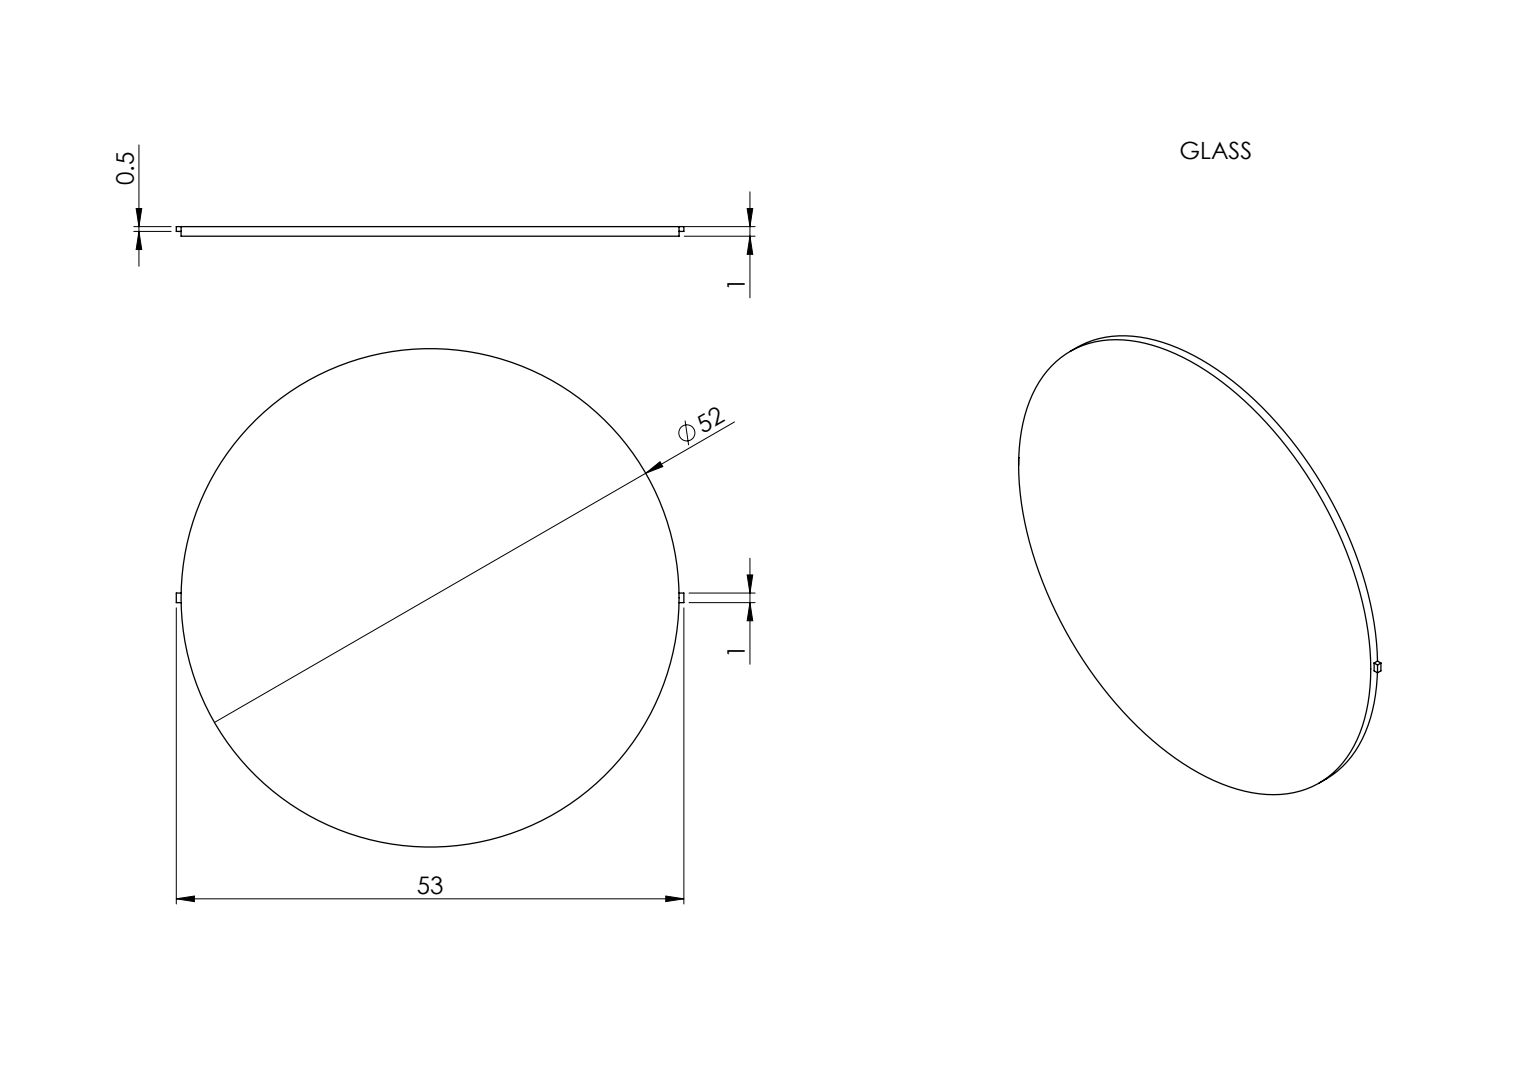
ISO-10303-21;
HEADER;
FILE_DESCRIPTION (('STEP AP214'),
    '1' );
FILE_NAME ('glass.step',
    '2026-10-26T12:50:16',
    ( '' ),
    ( '' ),
    'SwSTEP 2.0',
    'SolidWorks 2026',
    '' );
FILE_SCHEMA (( 'AUTOMOTIVE_DESIGN' ));
ENDSEC;

DATA;
#165=DIRECTION ( 'NONE',  ( -1.000000000000000000, 0.000000000000000000, 0.000000000000000000 ) ) ;
#175=LINE ( 'NONE', #12048, #20896 ) ;
#192=DIRECTION ( 'NONE',  ( 1.000000000000000000, -0.000000000000000000, -0.000000000000000000 ) ) ;
#288=ORIENTED_EDGE ( 'NONE', *, *, #23099, .T. ) ;
#324=DIRECTION ( 'NONE',  ( 0.000000000000000000, 0.000000000000000000, 1.000000000000000000 ) ) ;
#385=PLANE ( 'NONE',  #17255 ) ;
#447=LINE ( 'NONE', #10230, #15448 ) ;
#469=PRODUCT_DEFINITION_SHAPE ( 'NONE', 'NONE',  #20341 ) ;
#537=CARTESIAN_POINT ( 'NONE',  ( 0.000000000000000000, 0.000000000000000000, 19.50000000000000000 ) ) ;
#545=EDGE_LOOP ( 'NONE', ( #9181, #12765, #6775, #14139, #18806, #21870, #16789, #2419 ) ) ;
#649=EDGE_CURVE ( 'NONE', #12662, #14524, #9982, .T. ) ;
#747=FACE_OUTER_BOUND ( 'NONE', #11528, .T. ) ;
#913=CARTESIAN_POINT ( 'NONE',  ( 0.000000000000000000, 0.000000000000000000, 19.50000000000000000 ) ) ;
#940=CARTESIAN_POINT ( 'NONE',  ( 26.00000000000000711, 3.184081677783118980E-15, 20.00000000000000000 ) ) ;
#1040=UNCERTAINTY_MEASURE_WITH_UNIT (LENGTH_MEASURE( 1.000000000000000082E-05 ), #9039, 'distance_accuracy_value', 'NONE');
#1120=SHAPE_REPRESENTATION ( 'glass', ( #21036 ), #9344 ) ;
#1143=VERTEX_POINT ( 'NONE', #18649 ) ;
#1293=FACE_OUTER_BOUND ( 'NONE', #4147, .T. ) ;
#1406=ORIENTED_EDGE ( 'NONE', *, *, #3935, .F. ) ;
#1449=DIRECTION ( 'NONE',  ( 1.000000000000000000, 0.000000000000000000, 0.000000000000000000 ) ) ;
#1471=ADVANCED_FACE ( 'NONE', ( #20804 ), #3026, .T. ) ;
#1490=VECTOR ( 'NONE', #192, 1000.000000000000000 ) ;
#1528=VERTEX_POINT ( 'NONE', #940 ) ;
#1675=VECTOR ( 'NONE', #6954, 1000.000000000000000 ) ;
#1798=EDGE_CURVE ( 'NONE', #14524, #18045, #15690, .T. ) ;
#1814=DIRECTION ( 'NONE',  ( 1.000000000000000000, 0.000000000000000000, 0.000000000000000000 ) ) ;
#1866=ORIENTED_EDGE ( 'NONE', *, *, #3698, .F. ) ;
#1987=ORIENTED_EDGE ( 'NONE', *, *, #23515, .F. ) ;
#1995=AXIS2_PLACEMENT_3D ( 'NONE', #7561, #7812, #17496 ) ;
#2025=DIRECTION ( 'NONE',  ( 0.000000000000000000, 0.000000000000000000, -1.000000000000000000 ) ) ;
#2132=DIRECTION ( 'NONE',  ( -0.000000000000000000, -0.000000000000000000, -1.000000000000000000 ) ) ;
#2291=CARTESIAN_POINT ( 'NONE',  ( -26.50000000000000355, -0.5000000000000000000, 19.50000000000000000 ) ) ;
#2344=CARTESIAN_POINT ( 'NONE',  ( 26.49999999999999645, -0.5000000000000000000, 19.50000000000000000 ) ) ;
#2419=ORIENTED_EDGE ( 'NONE', *, *, #19939, .T. ) ;
#2431=CARTESIAN_POINT ( 'NONE',  ( 26.49999999999999645, -0.5000000000000000000, 19.50000000000000000 ) ) ;
#2446=FACE_OUTER_BOUND ( 'NONE', #24906, .T. ) ;
#2562=CARTESIAN_POINT ( 'NONE',  ( -25.99519186311192342, -0.5000000000000000000, 20.00000000000000000 ) ) ;
#2641=DIRECTION ( 'NONE',  ( 0.000000000000000000, 0.000000000000000000, -1.000000000000000000 ) ) ;
#2708=PLANE ( 'NONE',  #24311 ) ;
#2748=EDGE_LOOP ( 'NONE', ( #1866, #288, #10492, #1406 ) ) ;
#2946=ORIENTED_EDGE ( 'NONE', *, *, #3698, .T. ) ;
#2961=AXIS2_PLACEMENT_3D ( 'NONE', #23328, #5419, #13403 ) ;
#3026=PLANE ( 'NONE',  #8587 ) ;
#3046=ORIENTED_EDGE ( 'NONE', *, *, #23099, .F. ) ;
#3127=PRODUCT_DEFINITION_CONTEXT ( 'detailed design', #17969, 'design' ) ;
#3309=ADVANCED_FACE ( 'NONE', ( #15355 ), #17448, .T. ) ;
#3357=DIRECTION ( 'NONE',  ( 1.000000000000000000, -0.000000000000000000, -0.000000000000000000 ) ) ;
#3363=EDGE_LOOP ( 'NONE', ( #4654, #16710, #12568, #23853 ) ) ;
#3419=CIRCLE ( 'NONE', #21787, 26.00000000000000711 ) ;
#3496=COLOUR_RGB ( '',0.8941176470588234615, 0.8941176470588234615, 0.8941176470588234615 ) ;
#3606=EDGE_CURVE ( 'NONE', #12662, #13377, #25458, .T. ) ;
#3698=EDGE_CURVE ( 'NONE', #17369, #9796, #12489, .T. ) ;
#3751=APPLICATION_CONTEXT ( 'automotive_design' ) ;
#3754=LINE ( 'NONE', #23759, #24633 ) ;
#3796=ADVANCED_BREP_SHAPE_REPRESENTATION ( '', ( #22081, #21036 ), #9344 ) ;
#3851=DIRECTION ( 'NONE',  ( -0.000000000000000000, -0.000000000000000000, -1.000000000000000000 ) ) ;
#3877=CARTESIAN_POINT ( 'NONE',  ( 26.49999999999999645, 0.5000000000000000000, 19.00000000000000000 ) ) ;
#3924=( NAMED_UNIT ( * ) SI_UNIT ( $, .STERADIAN. ) SOLID_ANGLE_UNIT ( ) );
#3935=EDGE_CURVE ( 'NONE', #9796, #25585, #21733, .T. ) ;
#3948=VERTEX_POINT ( 'NONE', #18206 ) ;
#3953=ORIENTED_EDGE ( 'NONE', *, *, #19939, .F. ) ;
#3965=CARTESIAN_POINT ( 'NONE',  ( -26.50000000000000355, -0.5000000000000000000, 19.50000000000000000 ) ) ;
#3987=LINE ( 'NONE', #7781, #11324 ) ;
#4024=LINE ( 'NONE', #24681, #14557 ) ;
#4088=EDGE_CURVE ( 'NONE', #12917, #3948, #6942, .T. ) ;
#4147=EDGE_LOOP ( 'NONE', ( #25523, #16815, #25214, #3046, #1987 ) ) ;
#4355=EDGE_CURVE ( 'NONE', #14319, #1528, #8453, .T. ) ;
#4397=AXIS2_PLACEMENT_3D ( 'NONE', #22487, #16493, #10978 ) ;
#4414=CARTESIAN_POINT ( 'NONE',  ( 0.000000000000000000, 0.000000000000000000, 20.00000000000000000 ) ) ;
#4416=VERTEX_POINT ( 'NONE', #15955 ) ;
#4426=PRODUCT ( 'glass', 'glass', '', ( #9094 ) ) ;
#4554=DIRECTION ( 'NONE',  ( 0.000000000000000000, 0.000000000000000000, 1.000000000000000000 ) ) ;
#4654=ORIENTED_EDGE ( 'NONE', *, *, #5596, .F. ) ;
#4710=ADVANCED_FACE ( 'NONE', ( #12925 ), #385, .T. ) ;
#4936=ADVANCED_FACE ( 'NONE', ( #14981 ), #5044, .T. ) ;
#5044=CYLINDRICAL_SURFACE ( 'NONE', #21856, 26.00000000000000711 ) ;
#5078=ORIENTED_EDGE ( 'NONE', *, *, #24234, .T. ) ;
#5195=DIRECTION ( 'NONE',  ( 0.000000000000000000, 1.000000000000000000, 0.000000000000000000 ) ) ;
#5419=DIRECTION ( 'NONE',  ( 0.000000000000000000, 0.000000000000000000, 1.000000000000000000 ) ) ;
#5518=ORIENTED_EDGE ( 'NONE', *, *, #22622, .F. ) ;
#5596=EDGE_CURVE ( 'NONE', #18495, #14524, #8497, .T. ) ;
#5615=CARTESIAN_POINT ( 'NONE',  ( -25.99519186311192342, -0.5000000000000000000, 19.50000000000000000 ) ) ;
#5698=EDGE_LOOP ( 'NONE', ( #23371, #24133, #23127, #7405 ) ) ;
#5735=EDGE_CURVE ( 'NONE', #18705, #18585, #20613, .T. ) ;
#5943=DIRECTION ( 'NONE',  ( -1.000000000000000000, 0.000000000000000000, 0.000000000000000000 ) ) ;
#6028=CARTESIAN_POINT ( 'NONE',  ( 0.000000000000000000, 0.000000000000000000, 19.00000000000000000 ) ) ;
#6198=EDGE_CURVE ( 'NONE', #1528, #14319, #20521, .T. ) ;
#6268=( NAMED_UNIT ( * ) PLANE_ANGLE_UNIT ( ) SI_UNIT ( $, .RADIAN. ) );
#6284=DIRECTION ( 'NONE',  ( 0.000000000000000000, 0.000000000000000000, 1.000000000000000000 ) ) ;
#6352=ORIENTED_EDGE ( 'NONE', *, *, #22188, .T. ) ;
#6462=DIRECTION ( 'NONE',  ( 0.000000000000000000, 0.000000000000000000, 1.000000000000000000 ) ) ;
#6503=DIRECTION ( 'NONE',  ( -0.000000000000000000, -0.000000000000000000, -1.000000000000000000 ) ) ;
#6582=VECTOR ( 'NONE', #13913, 1000.000000000000000 ) ;
#6674=CARTESIAN_POINT ( 'NONE',  ( 25.99519186311192342, 0.5000000000000000000, 20.00000000000000000 ) ) ;
#6748=DIRECTION ( 'NONE',  ( 0.000000000000000000, 0.000000000000000000, -1.000000000000000000 ) ) ;
#6763=DIRECTION ( 'NONE',  ( 0.000000000000000000, -0.000000000000000000, 1.000000000000000000 ) ) ;
#6775=ORIENTED_EDGE ( 'NONE', *, *, #15340, .T. ) ;
#6842=DIRECTION ( 'NONE',  ( 0.000000000000000000, 0.000000000000000000, 1.000000000000000000 ) ) ;
#6891=PLANE ( 'NONE',  #16754 ) ;
#6912=SURFACE_STYLE_USAGE ( .BOTH. , #15024 ) ;
#6917=DIRECTION ( 'NONE',  ( 1.000000000000000000, 0.000000000000000000, 0.000000000000000000 ) ) ;
#6942=LINE ( 'NONE', #6674, #16399 ) ;
#6954=DIRECTION ( 'NONE',  ( 1.000000000000000000, -0.000000000000000000, -0.000000000000000000 ) ) ;
#6964=FACE_OUTER_BOUND ( 'NONE', #545, .T. ) ;
#7023=ORIENTED_EDGE ( 'NONE', *, *, #8660, .F. ) ;
#7072=( NAMED_UNIT ( * ) SI_UNIT ( $, .STERADIAN. ) SOLID_ANGLE_UNIT ( ) );
#7172=VECTOR ( 'NONE', #22696, 1000.000000000000000 ) ;
#7218=CARTESIAN_POINT ( 'NONE',  ( -26.00000000000000711, 0.000000000000000000, 19.50000000000000000 ) ) ;
#7405=ORIENTED_EDGE ( 'NONE', *, *, #3606, .T. ) ;
#7449=DIRECTION ( 'NONE',  ( 0.000000000000000000, 0.000000000000000000, 1.000000000000000000 ) ) ;
#7510=EDGE_LOOP ( 'NONE', ( #9564, #14844, #17583, #10328, #2946, #5078, #10015, #14168 ) ) ;
#7542=DIRECTION ( 'NONE',  ( 0.000000000000000000, 0.000000000000000000, -1.000000000000000000 ) ) ;
#7561=CARTESIAN_POINT ( 'NONE',  ( 0.000000000000000000, 0.000000000000000000, 19.50000000000000000 ) ) ;
#7563=CARTESIAN_POINT ( 'NONE',  ( 26.49999999999999645, -0.5000000000000000000, 19.50000000000000000 ) ) ;
#7656=LINE ( 'NONE', #13666, #1675 ) ;
#7781=CARTESIAN_POINT ( 'NONE',  ( -26.50000000000000355, -0.5000000000000000000, 19.50000000000000000 ) ) ;
#7789=CARTESIAN_POINT ( 'NONE',  ( 26.49999999999999645, -0.5000000000000000000, 19.50000000000000000 ) ) ;
#7812=DIRECTION ( 'NONE',  ( 0.000000000000000000, -0.000000000000000000, 1.000000000000000000 ) ) ;
#7880=CARTESIAN_POINT ( 'NONE',  ( -26.50000000000000355, -0.5000000000000000000, 19.00000000000000000 ) ) ;
#8107=ORIENTED_EDGE ( 'NONE', *, *, #22188, .F. ) ;
#8179=LINE ( 'NONE', #16156, #7172 ) ;
#8237=DIRECTION ( 'NONE',  ( -1.000000000000000000, 0.000000000000000000, 0.000000000000000000 ) ) ;
#8297=DIRECTION ( 'NONE',  ( 1.000000000000000000, 0.000000000000000000, 0.000000000000000000 ) ) ;
#8306=AXIS2_PLACEMENT_3D ( 'NONE', #4414, #6503, #16329 ) ;
#8431=DIRECTION ( 'NONE',  ( 1.000000000000000000, 0.000000000000000000, 0.000000000000000000 ) ) ;
#8453=CIRCLE ( 'NONE', #15547, 26.00000000000000711 ) ;
#8474=CARTESIAN_POINT ( 'NONE',  ( 26.49999999999999645, 0.5000000000000000000, 19.50000000000000000 ) ) ;
#8497=LINE ( 'NONE', #22867, #21044 ) ;
#8516=CARTESIAN_POINT ( 'NONE',  ( 25.99519186311192342, -0.5000000000000000000, 20.00000000000000000 ) ) ;
#8587=AXIS2_PLACEMENT_3D ( 'NONE', #10469, #16765, #2641 ) ;
#8590=EDGE_CURVE ( 'NONE', #3948, #18495, #14736, .T. ) ;
#8644=DIRECTION ( 'NONE',  ( -0.000000000000000000, -0.000000000000000000, -1.000000000000000000 ) ) ;
#8660=EDGE_CURVE ( 'NONE', #10164, #4416, #24575, .T. ) ;
#8688=CARTESIAN_POINT ( 'NONE',  ( 26.49999999999999645, -0.5000000000000000000, 19.00000000000000000 ) ) ;
#8717=DIRECTION ( 'NONE',  ( 0.000000000000000000, -0.000000000000000000, 1.000000000000000000 ) ) ;
#8888=( NAMED_UNIT ( * ) SI_UNIT ( $, .STERADIAN. ) SOLID_ANGLE_UNIT ( ) );
#8946=ORIENTED_EDGE ( 'NONE', *, *, #25469, .F. ) ;
#9039=( LENGTH_UNIT ( ) NAMED_UNIT ( * ) SI_UNIT ( .MILLI., .METRE. ) );
#9094=PRODUCT_CONTEXT ( 'NONE', #3751, 'mechanical' ) ;
#9112=ORIENTED_EDGE ( 'NONE', *, *, #10025, .F. ) ;
#9181=ORIENTED_EDGE ( 'NONE', *, *, #24234, .F. ) ;
#9235=SHAPE_DEFINITION_REPRESENTATION ( #469, #1120 ) ;
#9344=( GEOMETRIC_REPRESENTATION_CONTEXT ( 3 ) GLOBAL_UNCERTAINTY_ASSIGNED_CONTEXT ( ( #20656 ) ) GLOBAL_UNIT_ASSIGNED_CONTEXT ( ( #24180, #6268, #3924 ) ) REPRESENTATION_CONTEXT ( 'NONE', 'WORKASPACE' ) );
#9564=ORIENTED_EDGE ( 'NONE', *, *, #11490, .F. ) ;
#9796=VERTEX_POINT ( 'NONE', #14422 ) ;
#9886=CARTESIAN_POINT ( 'NONE',  ( -26.50000000000000355, 0.5000000000000000000, 19.50000000000000000 ) ) ;
#9982=LINE ( 'NONE', #16020, #1490 ) ;
#10015=ORIENTED_EDGE ( 'NONE', *, *, #8660, .T. ) ;
#10025=EDGE_CURVE ( 'NONE', #4416, #1143, #10887, .T. ) ;
#10128=AXIS2_PLACEMENT_3D ( 'NONE', #6028, #6284, #20666 ) ;
#10164=VERTEX_POINT ( 'NONE', #21296 ) ;
#10230=CARTESIAN_POINT ( 'NONE',  ( 26.49999999999999645, 0.5000000000000000000, 19.50000000000000000 ) ) ;
#10300=DIRECTION ( 'NONE',  ( 0.000000000000000000, 0.000000000000000000, -1.000000000000000000 ) ) ;
#10307=LINE ( 'NONE', #17794, #23006 ) ;
#10328=ORIENTED_EDGE ( 'NONE', *, *, #23515, .T. ) ;
#10362=CARTESIAN_POINT ( 'NONE',  ( 0.000000000000000000, 0.000000000000000000, 20.00000000000000000 ) ) ;
#10413=CYLINDRICAL_SURFACE ( 'NONE', #8306, 26.00000000000000711 ) ;
#10469=CARTESIAN_POINT ( 'NONE',  ( 26.49999999999999645, -0.5000000000000000000, 19.50000000000000000 ) ) ;
#10492=ORIENTED_EDGE ( 'NONE', *, *, #24097, .T. ) ;
#10536=VECTOR ( 'NONE', #22491, 1000.000000000000000 ) ;
#10577=MECHANICAL_DESIGN_GEOMETRIC_PRESENTATION_REPRESENTATION('',(#18128),#13936);
#10876=DIRECTION ( 'NONE',  ( 1.000000000000000000, -0.000000000000000000, -0.000000000000000000 ) ) ;
#10887=CIRCLE ( 'NONE', #24258, 26.00000000000000711 ) ;
#10978=DIRECTION ( 'NONE',  ( 1.000000000000000000, 0.000000000000000000, 0.000000000000000000 ) ) ;
#11022=ADVANCED_FACE ( 'NONE', ( #747 ), #6891, .T. ) ;
#11084=ADVANCED_FACE ( 'NONE', ( #2446 ), #24933, .T. ) ;
#11088=FILL_AREA_STYLE_COLOUR ( '', #3496 ) ;
#11324=VECTOR ( 'NONE', #2025, 1000.000000000000000 ) ;
#11465=EDGE_LOOP ( 'NONE', ( #7023, #3953, #22917, #6352 ) ) ;
#11490=EDGE_CURVE ( 'NONE', #1528, #1143, #8179, .T. ) ;
#11528=EDGE_LOOP ( 'NONE', ( #24469, #13562, #15601, #25845 ) ) ;
#11558=ORIENTED_EDGE ( 'NONE', *, *, #6198, .F. ) ;
#11570=CARTESIAN_POINT ( 'NONE',  ( -25.99519186311192342, 0.5000000000000000000, 19.50000000000000000 ) ) ;
#11853=ORIENTED_EDGE ( 'NONE', *, *, #5596, .T. ) ;
#12048=CARTESIAN_POINT ( 'NONE',  ( -26.00000000000000711, 0.000000000000000000, 20.00000000000000000 ) ) ;
#12470=PLANE ( 'NONE',  #16804 ) ;
#12489=LINE ( 'NONE', #2562, #22999 ) ;
#12527=VECTOR ( 'NONE', #10876, 1000.000000000000000 ) ;
#12565=EDGE_LOOP ( 'NONE', ( #21356, #24196 ) ) ;
#12568=ORIENTED_EDGE ( 'NONE', *, *, #3606, .F. ) ;
#12653=DIRECTION ( 'NONE',  ( 0.000000000000000000, -0.000000000000000000, 1.000000000000000000 ) ) ;
#12662=VERTEX_POINT ( 'NONE', #25605 ) ;
#12765=ORIENTED_EDGE ( 'NONE', *, *, #3935, .T. ) ;
#12777=CARTESIAN_POINT ( 'NONE',  ( 26.49999999999999645, 0.5000000000000000000, 19.50000000000000000 ) ) ;
#12907=DIRECTION ( 'NONE',  ( 1.000000000000000000, 0.000000000000000000, -0.000000000000000000 ) ) ;
#12917=VERTEX_POINT ( 'NONE', #18155 ) ;
#12925=FACE_OUTER_BOUND ( 'NONE', #17560, .T. ) ;
#13026=CARTESIAN_POINT ( 'NONE',  ( 0.000000000000000000, 0.000000000000000000, 20.00000000000000000 ) ) ;
#13138=PRODUCT_DEFINITION_FORMATION_WITH_SPECIFIED_SOURCE ( 'ANY', '', #4426, .NOT_KNOWN. ) ;
#13223=DIRECTION ( 'NONE',  ( 1.000000000000000000, 0.000000000000000000, 0.000000000000000000 ) ) ;
#13295=AXIS2_PLACEMENT_3D ( 'NONE', #537, #18689, #16490 ) ;
#13314=EDGE_CURVE ( 'NONE', #13377, #18495, #7656, .T. ) ;
#13353=CARTESIAN_POINT ( 'NONE',  ( 0.000000000000000000, 0.000000000000000000, 0.000000000000000000 ) ) ;
#13377=VERTEX_POINT ( 'NONE', #24745 ) ;
#13383=LINE ( 'NONE', #25668, #16838 ) ;
#13392=VECTOR ( 'NONE', #21196, 1000.000000000000000 ) ;
#13403=DIRECTION ( 'NONE',  ( 1.000000000000000000, 0.000000000000000000, -0.000000000000000000 ) ) ;
#13560=DIRECTION ( 'NONE',  ( 0.000000000000000000, -1.000000000000000000, -0.000000000000000000 ) ) ;
#13562=ORIENTED_EDGE ( 'NONE', *, *, #20462, .T. ) ;
#13666=CARTESIAN_POINT ( 'NONE',  ( 26.49999999999999645, 0.5000000000000000000, 19.00000000000000000 ) ) ;
#13675=DIRECTION ( 'NONE',  ( 0.000000000000000000, 0.000000000000000000, -1.000000000000000000 ) ) ;
#13913=DIRECTION ( 'NONE',  ( 0.000000000000000000, 1.000000000000000000, 0.000000000000000000 ) ) ;
#13936=( GEOMETRIC_REPRESENTATION_CONTEXT ( 3 ) GLOBAL_UNCERTAINTY_ASSIGNED_CONTEXT ( ( #22754 ) ) GLOBAL_UNIT_ASSIGNED_CONTEXT ( ( #14774, #18950, #8888 ) ) REPRESENTATION_CONTEXT ( 'NONE', 'WORKASPACE' ) );
#14139=ORIENTED_EDGE ( 'NONE', *, *, #13314, .T. ) ;
#14146=CARTESIAN_POINT ( 'NONE',  ( 26.49999999999999645, -0.5000000000000000000, 19.00000000000000000 ) ) ;
#14168=ORIENTED_EDGE ( 'NONE', *, *, #10025, .T. ) ;
#14169=DIRECTION ( 'NONE',  ( 0.000000000000000000, 0.000000000000000000, -1.000000000000000000 ) ) ;
#14319=VERTEX_POINT ( 'NONE', #24418 ) ;
#14422=CARTESIAN_POINT ( 'NONE',  ( -25.99519186311192342, -0.5000000000000000000, 19.00000000000000000 ) ) ;
#14510=DIRECTION ( 'NONE',  ( 0.000000000000000000, -0.000000000000000000, 1.000000000000000000 ) ) ;
#14524=VERTEX_POINT ( 'NONE', #11570 ) ;
#14557=VECTOR ( 'NONE', #5195, 1000.000000000000000 ) ;
#14639=CLOSED_SHELL ( 'NONE', ( #4936, #19694, #3309, #20551, #4710, #11084, #11022, #1471, #14819, #19714, #24870, #24317 ) ) ;
#14662=ORIENTED_EDGE ( 'NONE', *, *, #5735, .T. ) ;
#14722=DIRECTION ( 'NONE',  ( -1.000000000000000000, 0.000000000000000000, 0.000000000000000000 ) ) ;
#14736=CIRCLE ( 'NONE', #10128, 26.00000000000000711 ) ;
#14774=( LENGTH_UNIT ( ) NAMED_UNIT ( * ) SI_UNIT ( .MILLI., .METRE. ) );
#14819=ADVANCED_FACE ( 'NONE', ( #1293 ), #19456, .T. ) ;
#14825=DIRECTION ( 'NONE',  ( 1.000000000000000000, 0.000000000000000000, -0.000000000000000000 ) ) ;
#14842=CARTESIAN_POINT ( 'NONE',  ( 0.000000000000000000, 0.000000000000000000, 19.00000000000000000 ) ) ;
#14844=ORIENTED_EDGE ( 'NONE', *, *, #4355, .F. ) ;
#14895=SHAPE_REPRESENTATION_RELATIONSHIP ( 'NONE' , 'NONE' ,  #1120, #3796 ) ;
#14981=FACE_OUTER_BOUND ( 'NONE', #18207, .T. ) ;
#15024=SURFACE_SIDE_STYLE ('',( #16871 ) ) ;
#15148=ORIENTED_EDGE ( 'NONE', *, *, #8590, .T. ) ;
#15172=CARTESIAN_POINT ( 'NONE',  ( -25.99519186311192342, 0.5000000000000000000, 19.00000000000000000 ) ) ;
#15340=EDGE_CURVE ( 'NONE', #25585, #13377, #25799, .T. ) ;
#15355=FACE_OUTER_BOUND ( 'NONE', #12565, .T. ) ;
#15414=CARTESIAN_POINT ( 'NONE',  ( 26.49999999999999645, -0.5000000000000000000, 19.00000000000000000 ) ) ;
#15448=VECTOR ( 'NONE', #14169, 1000.000000000000000 ) ;
#15547=AXIS2_PLACEMENT_3D ( 'NONE', #23033, #7449, #1449 ) ;
#15569=ORIENTED_EDGE ( 'NONE', *, *, #22944, .F. ) ;
#15601=ORIENTED_EDGE ( 'NONE', *, *, #20281, .T. ) ;
#15690=CIRCLE ( 'NONE', #4397, 26.00000000000000711 ) ;
#15703=DIRECTION ( 'NONE',  ( 0.000000000000000000, 0.000000000000000000, 1.000000000000000000 ) ) ;
#15955=CARTESIAN_POINT ( 'NONE',  ( 25.99519186311192342, -0.5000000000000000000, 19.50000000000000000 ) ) ;
#16020=CARTESIAN_POINT ( 'NONE',  ( 26.49999999999999645, 0.5000000000000000000, 19.50000000000000000 ) ) ;
#16056=DIRECTION ( 'NONE',  ( -1.000000000000000000, 0.000000000000000000, 0.000000000000000000 ) ) ;
#16156=CARTESIAN_POINT ( 'NONE',  ( 26.00000000000000711, 3.184081677783118980E-15, 20.00000000000000000 ) ) ;
#16329=DIRECTION ( 'NONE',  ( -1.000000000000000000, 0.000000000000000000, 0.000000000000000000 ) ) ;
#16344=AXIS2_PLACEMENT_3D ( 'NONE', #16966, #6763, #12907 ) ;
#16399=VECTOR ( 'NONE', #8644, 1000.000000000000000 ) ;
#16451=VECTOR ( 'NONE', #6748, 1000.000000000000000 ) ;
#16459=FACE_OUTER_BOUND ( 'NONE', #3363, .T. ) ;
#16474=EDGE_CURVE ( 'NONE', #24372, #12662, #4024, .T. ) ;
#16490=DIRECTION ( 'NONE',  ( 1.000000000000000000, 0.000000000000000000, 0.000000000000000000 ) ) ;
#16493=DIRECTION ( 'NONE',  ( 0.000000000000000000, -0.000000000000000000, 1.000000000000000000 ) ) ;
#16512=CARTESIAN_POINT ( 'NONE',  ( -26.50000000000000355, -0.5000000000000000000, 19.00000000000000000 ) ) ;
#16577=CARTESIAN_POINT ( 'NONE',  ( 26.49999999999999645, 0.5000000000000000000, 19.50000000000000000 ) ) ;
#16710=ORIENTED_EDGE ( 'NONE', *, *, #13314, .F. ) ;
#16733=PRESENTATION_STYLE_ASSIGNMENT (( #6912 ) ) ;
#16754=AXIS2_PLACEMENT_3D ( 'NONE', #8474, #20883, #8717 ) ;
#16765=DIRECTION ( 'NONE',  ( 0.000000000000000000, -1.000000000000000000, -0.000000000000000000 ) ) ;
#16789=ORIENTED_EDGE ( 'NONE', *, *, #25469, .T. ) ;
#16790=PLANE ( 'NONE',  #17133 ) ;
#16804=AXIS2_PLACEMENT_3D ( 'NONE', #2291, #24634, #324 ) ;
#16813=FACE_OUTER_BOUND ( 'NONE', #5698, .T. ) ;
#16815=ORIENTED_EDGE ( 'NONE', *, *, #649, .F. ) ;
#16838=VECTOR ( 'NONE', #25398, 1000.000000000000000 ) ;
#16871=SURFACE_STYLE_FILL_AREA ( #24445 ) ;
#16966=CARTESIAN_POINT ( 'NONE',  ( 0.000000000000000000, 0.000000000000000000, 19.50000000000000000 ) ) ;
#17038=ORIENTED_EDGE ( 'NONE', *, *, #20462, .F. ) ;
#17133=AXIS2_PLACEMENT_3D ( 'NONE', #22920, #6842, #14825 ) ;
#17156=CARTESIAN_POINT ( 'NONE',  ( 26.49999999999999645, -0.5000000000000000000, 19.50000000000000000 ) ) ;
#17255=AXIS2_PLACEMENT_3D ( 'NONE', #2344, #24555, #10300 ) ;
#17369=VERTEX_POINT ( 'NONE', #5615 ) ;
#17421=ORIENTED_EDGE ( 'NONE', *, *, #18449, .F. ) ;
#17448=PLANE ( 'NONE',  #2961 ) ;
#17496=DIRECTION ( 'NONE',  ( 1.000000000000000000, 0.000000000000000000, -0.000000000000000000 ) ) ;
#17533=STYLED_ITEM('',(#25900),#22081);
#17560=EDGE_LOOP ( 'NONE', ( #8946, #24612, #19493, #14662 ) ) ;
#17583=ORIENTED_EDGE ( 'NONE', *, *, #22622, .T. ) ;
#17737=PLANE ( 'NONE',  #22931 ) ;
#17757=CARTESIAN_POINT ( 'NONE',  ( 0.000000000000000000, 0.000000000000000000, 19.50000000000000000 ) ) ;
#17794=CARTESIAN_POINT ( 'NONE',  ( 26.49999999999999645, -0.5000000000000000000, 19.50000000000000000 ) ) ;
#17842=EDGE_CURVE ( 'NONE', #3948, #19738, #25330, .T. ) ;
#17882=DIRECTION ( 'NONE',  ( 0.000000000000000000, -0.000000000000000000, 1.000000000000000000 ) ) ;
#17969=APPLICATION_CONTEXT ( 'automotive_design' ) ;
#18045=VERTEX_POINT ( 'NONE', #7218 ) ;
#18128=STYLED_ITEM ( 'NONE', ( #16733 ), #3796 ) ;
#18138=CARTESIAN_POINT ( 'NONE',  ( 26.49999999999999645, 0.5000000000000000000, 19.00000000000000000 ) ) ;
#18155=CARTESIAN_POINT ( 'NONE',  ( 25.99519186311192342, 0.5000000000000000000, 19.50000000000000000 ) ) ;
#18177=ORIENTED_EDGE ( 'NONE', *, *, #1798, .T. ) ;
#18206=CARTESIAN_POINT ( 'NONE',  ( 25.99519186311192342, 0.5000000000000000000, 19.00000000000000000 ) ) ;
#18207=EDGE_LOOP ( 'NONE', ( #11558, #19024, #18765, #23685, #15148, #11853, #18177, #5518 ) ) ;
#18449=EDGE_CURVE ( 'NONE', #1143, #12917, #24559, .T. ) ;
#18495=VERTEX_POINT ( 'NONE', #15172 ) ;
#18585=VERTEX_POINT ( 'NONE', #15414 ) ;
#18649=CARTESIAN_POINT ( 'NONE',  ( 26.00000000000000711, 3.184081677783118980E-15, 19.50000000000000000 ) ) ;
#18689=DIRECTION ( 'NONE',  ( 0.000000000000000000, -0.000000000000000000, 1.000000000000000000 ) ) ;
#18705=VERTEX_POINT ( 'NONE', #7563 ) ;
#18765=ORIENTED_EDGE ( 'NONE', *, *, #18449, .T. ) ;
#18805=MECHANICAL_DESIGN_GEOMETRIC_PRESENTATION_REPRESENTATION('',(#17533),#22963);
#18806=ORIENTED_EDGE ( 'NONE', *, *, #8590, .F. ) ;
#18950=( NAMED_UNIT ( * ) PLANE_ANGLE_UNIT ( ) SI_UNIT ( $, .RADIAN. ) );
#19024=ORIENTED_EDGE ( 'NONE', *, *, #11490, .T. ) ;
#19456=PLANE ( 'NONE',  #1995 ) ;
#19493=ORIENTED_EDGE ( 'NONE', *, *, #22944, .T. ) ;
#19531=VECTOR ( 'NONE', #3357, 1000.000000000000000 ) ;
#19658=VECTOR ( 'NONE', #165, 1000.000000000000000 ) ;
#19694=ADVANCED_FACE ( 'NONE', ( #24541 ), #10413, .T. ) ;
#19714=ADVANCED_FACE ( 'NONE', ( #20072 ), #17737, .T. ) ;
#19738=VERTEX_POINT ( 'NONE', #18138 ) ;
#19939=EDGE_CURVE ( 'NONE', #18585, #10164, #24397, .T. ) ;
#20072=FACE_OUTER_BOUND ( 'NONE', #2748, .T. ) ;
#20079=CIRCLE ( 'NONE', #25526, 26.00000000000000711 ) ;
#20281=EDGE_CURVE ( 'NONE', #23846, #19738, #447, .T. ) ;
#20341=PRODUCT_DEFINITION ( 'UNKNOWN', '', #13138, #3127 ) ;
#20462=EDGE_CURVE ( 'NONE', #12917, #23846, #21211, .T. ) ;
#20521=CIRCLE ( 'NONE', #22189, 26.00000000000000711 ) ;
#20551=ADVANCED_FACE ( 'NONE', ( #6964 ), #16790, .F. ) ;
#20591=DIRECTION ( 'NONE',  ( 0.000000000000000000, 0.000000000000000000, 1.000000000000000000 ) ) ;
#20613=LINE ( 'NONE', #2431, #16451 ) ;
#20656=UNCERTAINTY_MEASURE_WITH_UNIT (LENGTH_MEASURE( 1.000000000000000082E-05 ), #24180, 'distance_accuracy_value', 'NONE');
#20666=DIRECTION ( 'NONE',  ( 1.000000000000000000, 0.000000000000000000, 0.000000000000000000 ) ) ;
#20804=FACE_OUTER_BOUND ( 'NONE', #11465, .T. ) ;
#20883=DIRECTION ( 'NONE',  ( 0.000000000000000000, 1.000000000000000000, 0.000000000000000000 ) ) ;
#20896=VECTOR ( 'NONE', #2132, 1000.000000000000000 ) ;
#21036=AXIS2_PLACEMENT_3D ( 'NONE', #13353, #15703, #13223 ) ;
#21044=VECTOR ( 'NONE', #4554, 1000.000000000000000 ) ;
#21196=DIRECTION ( 'NONE',  ( -0.000000000000000000, -1.000000000000000000, -0.000000000000000000 ) ) ;
#21211=LINE ( 'NONE', #22797, #12527 ) ;
#21285=VECTOR ( 'NONE', #14722, 1000.000000000000000 ) ;
#21296=CARTESIAN_POINT ( 'NONE',  ( 25.99519186311192342, -0.5000000000000000000, 19.00000000000000000 ) ) ;
#21356=ORIENTED_EDGE ( 'NONE', *, *, #4355, .T. ) ;
#21733=LINE ( 'NONE', #14146, #19658 ) ;
#21787=AXIS2_PLACEMENT_3D ( 'NONE', #14842, #20591, #8297 ) ;
#21856=AXIS2_PLACEMENT_3D ( 'NONE', #13026, #3851, #5943 ) ;
#21870=ORIENTED_EDGE ( 'NONE', *, *, #17842, .T. ) ;
#22081=MANIFOLD_SOLID_BREP ( 'Boss-Extrude2', #14639 ) ;
#22182=DIRECTION ( 'NONE',  ( -0.000000000000000000, -0.000000000000000000, -1.000000000000000000 ) ) ;
#22188=EDGE_CURVE ( 'NONE', #18705, #4416, #3754, .T. ) ;
#22189=AXIS2_PLACEMENT_3D ( 'NONE', #10362, #6462, #8431 ) ;
#22487=CARTESIAN_POINT ( 'NONE',  ( 0.000000000000000000, 0.000000000000000000, 19.50000000000000000 ) ) ;
#22491=DIRECTION ( 'NONE',  ( 0.000000000000000000, 0.000000000000000000, 1.000000000000000000 ) ) ;
#22622=EDGE_CURVE ( 'NONE', #14319, #18045, #175, .T. ) ;
#22696=DIRECTION ( 'NONE',  ( -0.000000000000000000, -0.000000000000000000, -1.000000000000000000 ) ) ;
#22754=UNCERTAINTY_MEASURE_WITH_UNIT (LENGTH_MEASURE( 1.000000000000000082E-05 ), #14774, 'distance_accuracy_value', 'NONE');
#22797=CARTESIAN_POINT ( 'NONE',  ( 26.49999999999999645, 0.5000000000000000000, 19.50000000000000000 ) ) ;
#22848=DIRECTION ( 'NONE',  ( 0.000000000000000000, 1.000000000000000000, 0.000000000000000000 ) ) ;
#22867=CARTESIAN_POINT ( 'NONE',  ( -25.99519186311192342, 0.5000000000000000000, 20.00000000000000000 ) ) ;
#22917=ORIENTED_EDGE ( 'NONE', *, *, #5735, .F. ) ;
#22920=CARTESIAN_POINT ( 'NONE',  ( 0.000000000000000000, 0.000000000000000000, 19.00000000000000000 ) ) ;
#22931=AXIS2_PLACEMENT_3D ( 'NONE', #7789, #13560, #13675 ) ;
#22944=EDGE_CURVE ( 'NONE', #23846, #18705, #25641, .T. ) ;
#22963=( GEOMETRIC_REPRESENTATION_CONTEXT ( 3 ) GLOBAL_UNCERTAINTY_ASSIGNED_CONTEXT ( ( #1040 ) ) GLOBAL_UNIT_ASSIGNED_CONTEXT ( ( #9039, #24987, #7072 ) ) REPRESENTATION_CONTEXT ( 'NONE', 'WORKASPACE' ) );
#22999=VECTOR ( 'NONE', #22182, 1000.000000000000000 ) ;
#23006=VECTOR ( 'NONE', #8237, 1000.000000000000000 ) ;
#23033=CARTESIAN_POINT ( 'NONE',  ( 0.000000000000000000, 0.000000000000000000, 20.00000000000000000 ) ) ;
#23099=EDGE_CURVE ( 'NONE', #17369, #24372, #10307, .T. ) ;
#23127=ORIENTED_EDGE ( 'NONE', *, *, #16474, .T. ) ;
#23328=CARTESIAN_POINT ( 'NONE',  ( 0.000000000000000000, 0.000000000000000000, 20.00000000000000000 ) ) ;
#23371=ORIENTED_EDGE ( 'NONE', *, *, #15340, .F. ) ;
#23515=EDGE_CURVE ( 'NONE', #18045, #17369, #20079, .T. ) ;
#23685=ORIENTED_EDGE ( 'NONE', *, *, #4088, .T. ) ;
#23759=CARTESIAN_POINT ( 'NONE',  ( 26.49999999999999645, -0.5000000000000000000, 19.50000000000000000 ) ) ;
#23846=VERTEX_POINT ( 'NONE', #12777 ) ;
#23853=ORIENTED_EDGE ( 'NONE', *, *, #649, .T. ) ;
#24097=EDGE_CURVE ( 'NONE', #24372, #25585, #3987, .T. ) ;
#24133=ORIENTED_EDGE ( 'NONE', *, *, #24097, .F. ) ;
#24180=( LENGTH_UNIT ( ) NAMED_UNIT ( * ) SI_UNIT ( .MILLI., .METRE. ) );
#24196=ORIENTED_EDGE ( 'NONE', *, *, #6198, .T. ) ;
#24234=EDGE_CURVE ( 'NONE', #9796, #10164, #3419, .T. ) ;
#24258=AXIS2_PLACEMENT_3D ( 'NONE', #913, #14510, #6917 ) ;
#24311=AXIS2_PLACEMENT_3D ( 'NONE', #16577, #22848, #12653 ) ;
#24317=ADVANCED_FACE ( 'NONE', ( #16813 ), #12470, .T. ) ;
#24372=VERTEX_POINT ( 'NONE', #3965 ) ;
#24397=LINE ( 'NONE', #8688, #21285 ) ;
#24418=CARTESIAN_POINT ( 'NONE',  ( -26.00000000000000711, 0.000000000000000000, 20.00000000000000000 ) ) ;
#24445=FILL_AREA_STYLE ('',( #11088 ) ) ;
#24469=ORIENTED_EDGE ( 'NONE', *, *, #4088, .F. ) ;
#24541=FACE_OUTER_BOUND ( 'NONE', #7510, .T. ) ;
#24555=DIRECTION ( 'NONE',  ( 1.000000000000000000, -0.000000000000000000, 0.000000000000000000 ) ) ;
#24559=CIRCLE ( 'NONE', #13295, 26.00000000000000711 ) ;
#24575=LINE ( 'NONE', #8516, #10536 ) ;
#24612=ORIENTED_EDGE ( 'NONE', *, *, #20281, .F. ) ;
#24633=VECTOR ( 'NONE', #16056, 1000.000000000000000 ) ;
#24634=DIRECTION ( 'NONE',  ( -1.000000000000000000, 0.000000000000000000, 0.000000000000000000 ) ) ;
#24663=VECTOR ( 'NONE', #7542, 1000.000000000000000 ) ;
#24681=CARTESIAN_POINT ( 'NONE',  ( -26.50000000000000355, -0.5000000000000000000, 19.50000000000000000 ) ) ;
#24745=CARTESIAN_POINT ( 'NONE',  ( -26.50000000000000355, 0.5000000000000000000, 19.00000000000000000 ) ) ;
#24870=ADVANCED_FACE ( 'NONE', ( #16459 ), #2708, .T. ) ;
#24906=EDGE_LOOP ( 'NONE', ( #9112, #8107, #15569, #17038, #17421 ) ) ;
#24933=PLANE ( 'NONE',  #16344 ) ;
#24987=( NAMED_UNIT ( * ) PLANE_ANGLE_UNIT ( ) SI_UNIT ( $, .RADIAN. ) );
#25214=ORIENTED_EDGE ( 'NONE', *, *, #16474, .F. ) ;
#25330=LINE ( 'NONE', #3877, #19531 ) ;
#25398=DIRECTION ( 'NONE',  ( -0.000000000000000000, -1.000000000000000000, -0.000000000000000000 ) ) ;
#25458=LINE ( 'NONE', #9886, #24663 ) ;
#25469=EDGE_CURVE ( 'NONE', #19738, #18585, #13383, .T. ) ;
#25523=ORIENTED_EDGE ( 'NONE', *, *, #1798, .F. ) ;
#25526=AXIS2_PLACEMENT_3D ( 'NONE', #17757, #17882, #1814 ) ;
#25585=VERTEX_POINT ( 'NONE', #16512 ) ;
#25605=CARTESIAN_POINT ( 'NONE',  ( -26.50000000000000355, 0.5000000000000000000, 19.50000000000000000 ) ) ;
#25641=LINE ( 'NONE', #17156, #13392 ) ;
#25668=CARTESIAN_POINT ( 'NONE',  ( 26.49999999999999645, -0.5000000000000000000, 19.00000000000000000 ) ) ;
#25799=LINE ( 'NONE', #7880, #6582 ) ;
#25845=ORIENTED_EDGE ( 'NONE', *, *, #17842, .F. ) ;
#25894=COLOUR_RGB('Light Blue',0.38,0.62,0.78);
#25895=FILL_AREA_STYLE_COLOUR('',#25894);
#25896=FILL_AREA_STYLE('',(#25895));
#25897=SURFACE_STYLE_FILL_AREA(#25896);
#25898=SURFACE_SIDE_STYLE('',(#25897));
#25899=SURFACE_STYLE_USAGE(.BOTH.,#25898);
#25900=PRESENTATION_STYLE_ASSIGNMENT((#25899));
ENDSEC;
END-ISO-10303-21;
